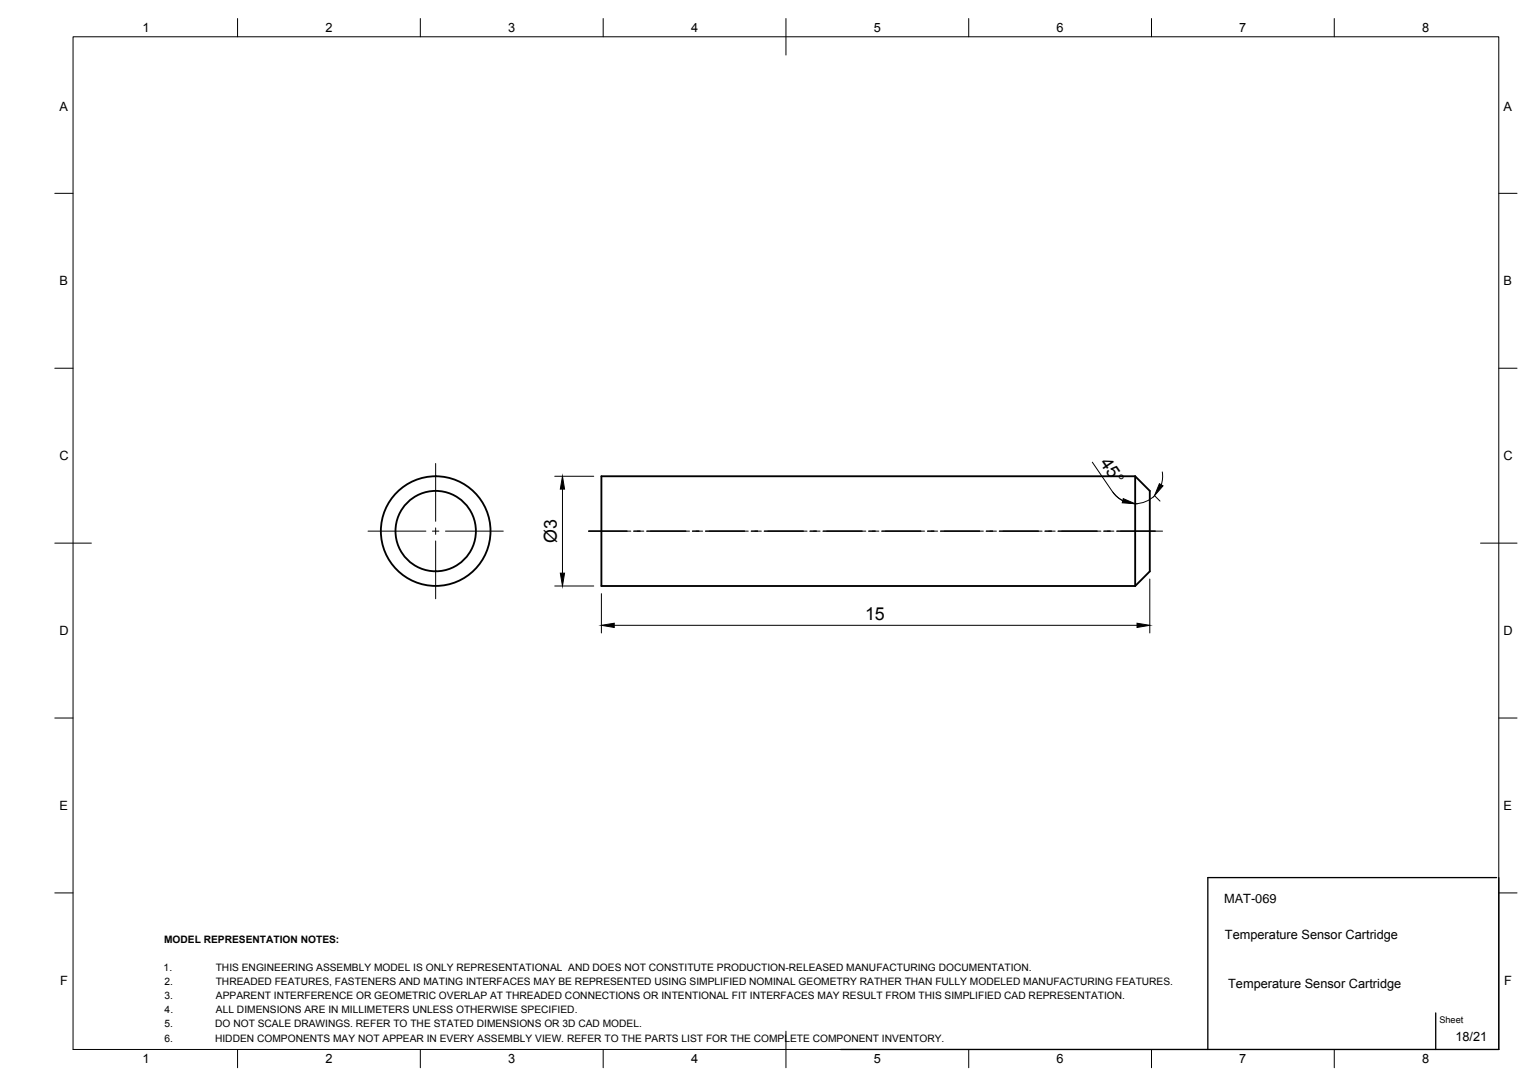
ISO-10303-21;
HEADER;
/* Generated by software containing ST-Developer
 * from STEP Tools, Inc. (www.steptools.com) 
 */

FILE_DESCRIPTION(
/* description */ ('CAx-IF Rec.Pracs.---Representation and Presentation of Product Manufa
cturing Information (PMI)---4.0---2014-10-13'),
/* implementation_level */ '2;1');

FILE_NAME(
/* name */ 'Temperature Sensor Cartridge.step',
/* time_stamp */ '2026-10-24T15:08:39-07:00',
/* author */ (''),
/* organization */ (''),
/* preprocessor_version */ 'ST-DEVELOPER v20.2',
/* originating_system */ 'Autodesk Translation Framework v15.17.0.0',
/* authorisation */ '');

FILE_SCHEMA (('AP242_MANAGED_MODEL_BASED_3D_ENGINEERING_MIM_LF { 1 0 10303 442 2 1 4 }'));
ENDSEC;

DATA;
#10=MECHANICAL_DESIGN_GEOMETRIC_PRESENTATION_REPRESENTATION('',(#835),#50081);
#654=CONICAL_SURFACE('',#10892,0.0013,0.785398163397448);
#795=SHAPE_REPRESENTATION_RELATIONSHIP('SRR','None',#50163,#815);
#815=ADVANCED_BREP_SHAPE_REPRESENTATION('',(#855),#50076);
#835=STYLED_ITEM('',(#50262),#855);
#855=MANIFOLD_SOLID_BREP('Body1',#9880);
#1083=PLANE('',#10897);
#1084=PLANE('',#10898);
#1562=FACE_OUTER_BOUND('',#2157,.T.);
#1563=FACE_OUTER_BOUND('',#2158,.T.);
#1564=FACE_OUTER_BOUND('',#2159,.T.);
#1565=FACE_OUTER_BOUND('',#2160,.T.);
#2157=EDGE_LOOP('',(#8760,#8761,#8762,#8763));
#2158=EDGE_LOOP('',(#8764,#8765,#8766,#8767));
#2159=EDGE_LOOP('',(#8768));
#2160=EDGE_LOOP('',(#8769));
#2764=LINE('',#45877,#3342);
#2765=LINE('',#45882,#3343);
#3342=VECTOR('',#13132,0.0013);
#3343=VECTOR('',#13139,0.0015);
#3730=CIRCLE('',#10893,0.00150000000001);
#3731=CIRCLE('',#10894,0.00110000000001);
#3732=CIRCLE('',#10896,0.00150000000001);
#4641=VERTEX_POINT('',#45874);
#4642=VERTEX_POINT('',#45876);
#4643=VERTEX_POINT('',#45880);
#6033=EDGE_CURVE('',#4641,#4641,#3730,.T.);
#6034=EDGE_CURVE('',#4641,#4642,#2764,.T.);
#6035=EDGE_CURVE('',#4642,#4642,#3731,.T.);
#6036=EDGE_CURVE('',#4643,#4643,#3732,.T.);
#6037=EDGE_CURVE('',#4643,#4641,#2765,.T.);
#8760=ORIENTED_EDGE('',*,*,#6033,.T.);
#8761=ORIENTED_EDGE('',*,*,#6034,.T.);
#8762=ORIENTED_EDGE('',*,*,#6035,.T.);
#8763=ORIENTED_EDGE('',*,*,#6034,.F.);
#8764=ORIENTED_EDGE('',*,*,#6036,.F.);
#8765=ORIENTED_EDGE('',*,*,#6037,.T.);
#8766=ORIENTED_EDGE('',*,*,#6033,.F.);
#8767=ORIENTED_EDGE('',*,*,#6037,.F.);
#8768=ORIENTED_EDGE('',*,*,#6035,.F.);
#8769=ORIENTED_EDGE('',*,*,#6036,.T.);
#9280=CYLINDRICAL_SURFACE('',#10895,0.0015);
#9784=ADVANCED_FACE('',(#1562),#654,.T.);
#9785=ADVANCED_FACE('',(#1563),#9280,.T.);
#9786=ADVANCED_FACE('',(#1564),#1083,.F.);
#9787=ADVANCED_FACE('',(#1565),#1084,.T.);
#9880=CLOSED_SHELL('',(#9784,#9785,#9786,#9787));
#10891=AXIS2_PLACEMENT_3D('',#45872,#13126,#13127);
#10892=AXIS2_PLACEMENT_3D('',#45873,#13128,#13129);
#10893=AXIS2_PLACEMENT_3D('',#45875,#13130,#13131);
#10894=AXIS2_PLACEMENT_3D('',#45878,#13133,#13134);
#10895=AXIS2_PLACEMENT_3D('',#45879,#13135,#13136);
#10896=AXIS2_PLACEMENT_3D('',#45881,#13137,#13138);
#10897=AXIS2_PLACEMENT_3D('',#45883,#13140,#13141);
#10898=AXIS2_PLACEMENT_3D('',#45884,#13142,#13143);
#13126=DIRECTION('axis',(0.,0.,1.));
#13127=DIRECTION('refdir',(1.,0.,0.));
#13128=DIRECTION('center_axis',(-2.42833204006769E-16,-2.41473507855972E-15,
1.));
#13129=DIRECTION('ref_axis',(0.422618261740706,0.906307787036647,2.29111895189949E-15));
#13130=DIRECTION('center_axis',(2.42833204006769E-16,2.41473507855972E-15,
-1.));
#13131=DIRECTION('ref_axis',(0.422618261740706,0.906307787036647,2.29111895189949E-15));
#13132=DIRECTION('',(0.298836238730124,0.640856382055788,-0.707106781186546));
#13133=DIRECTION('center_axis',(-2.42833204006769E-16,-2.41473507855972E-15,
1.));
#13134=DIRECTION('ref_axis',(0.422618261740706,0.906307787036647,2.29111895189949E-15));
#13135=DIRECTION('center_axis',(-2.42833204006769E-16,-2.41473507855972E-15,
1.));
#13136=DIRECTION('ref_axis',(0.422618261740706,0.906307787036647,2.29111895189949E-15));
#13137=DIRECTION('center_axis',(-2.42833204006769E-16,-2.41473507855972E-15,
1.));
#13138=DIRECTION('ref_axis',(0.422618261740706,0.906307787036647,2.29111895189949E-15));
#13139=DIRECTION('',(2.42833204006769E-16,2.41473507855972E-15,-1.));
#13140=DIRECTION('center_axis',(-2.42833204006769E-16,-2.41473507855972E-15,
1.));
#13141=DIRECTION('ref_axis',(0.422618261740706,0.906307787036647,2.29111895189949E-15));
#13142=DIRECTION('center_axis',(-2.42833204006769E-16,-2.41473507855972E-15,
1.));
#13143=DIRECTION('ref_axis',(0.422618261740706,0.906307787036647,2.29111895189949E-15));
#45872=CARTESIAN_POINT('',(0.,0.,0.));
#45873=CARTESIAN_POINT('Origin',(0.006,-0.0355287743898723,-0.0193758532865581));
#45874=CARTESIAN_POINT('',(0.00536607260738471,-0.0368882360704363,-0.0191758532865481));
#45875=CARTESIAN_POINT('Origin',(0.006,-0.0355287743898723,-0.0191758532865481));
#45876=CARTESIAN_POINT('',(0.00553511991208311,-0.0365257129556171,-0.0195758532865531));
#45877=CARTESIAN_POINT('',(0.00545059625973708,-0.0367069745130199,-0.0193758532865581));
#45878=CARTESIAN_POINT('Origin',(0.006,-0.0355287743898723,-0.0195758532865581));
#45879=CARTESIAN_POINT('Origin',(0.006,-0.0355287743898723,-0.0195758532865581));
#45880=CARTESIAN_POINT('',(0.00536607260738894,-0.0368882360704273,-0.0045758532865481));
#45881=CARTESIAN_POINT('Origin',(0.006,-0.0355287743898724,-0.0045758532865481));
#45882=CARTESIAN_POINT('',(0.00536607260738894,-0.0368882360704273,-0.0195758532865581));
#45883=CARTESIAN_POINT('Origin',(0.006,-0.0355287743898723,-0.0195758532865581));
#45884=CARTESIAN_POINT('Origin',(0.006,-0.0355287743898724,-0.0045758532865581));
#50054=UNCERTAINTY_MEASURE_WITH_UNIT(LENGTH_MEASURE(1.E-5),#50082,
'DISTANCE_ACCURACY_VALUE',
'Maximum model space distance between geometric entities at asserted c
onnectivities');
#50059=UNCERTAINTY_MEASURE_WITH_UNIT(LENGTH_MEASURE(1.E-5),#50082,
'DISTANCE_ACCURACY_VALUE',
'Maximum model space distance between geometric entities at asserted c
onnectivities');
#50076=(
GEOMETRIC_REPRESENTATION_CONTEXT(3)
GLOBAL_UNCERTAINTY_ASSIGNED_CONTEXT((#50054))
GLOBAL_UNIT_ASSIGNED_CONTEXT((#50082,#50083,#50084))
REPRESENTATION_CONTEXT('','3D')
);
#50081=(
GEOMETRIC_REPRESENTATION_CONTEXT(3)
GLOBAL_UNCERTAINTY_ASSIGNED_CONTEXT((#50059))
GLOBAL_UNIT_ASSIGNED_CONTEXT((#50082,#50083,#50084))
REPRESENTATION_CONTEXT('','3D')
);
#50082=(
LENGTH_UNIT()
NAMED_UNIT(*)
SI_UNIT($,.METRE.)
);
#50083=(
NAMED_UNIT(*)
PLANE_ANGLE_UNIT()
SI_UNIT($,.RADIAN.)
);
#50084=(
NAMED_UNIT(*)
SI_UNIT($,.STERADIAN.)
SOLID_ANGLE_UNIT()
);
#50101=SHAPE_DEFINITION_REPRESENTATION(#50122,#50163);
#50122=PRODUCT_DEFINITION_SHAPE('',$,#50185);
#50163=SHAPE_REPRESENTATION('',(#10891),#50076);
#50168=PRODUCT_DEFINITION_CONTEXT('part definition',#50233,'design');
#50185=PRODUCT_DEFINITION('Temperature Sensor Cartridge',
'Temperature Sensor Cartridge',#50206,#50168);
#50206=PRODUCT_DEFINITION_FORMATION('',$,#50251);
#50233=APPLICATION_CONTEXT('Managed model based 3d engineering');
#50234=PRODUCT_CONTEXT('part definition',#50233,'mechanical');
#50251=PRODUCT('Temperature Sensor Cartridge',
'Temperature Sensor Cartridge',
'LEGAL AND USAGE DISCLAIMER: this Data/Model is provided \X2\201C\X0\A
S IS\X2\201D\X0\ for informational and representational only. It is a 
geometric approximation and is NOT engineered, certified, or guarantee
d for dimensional accuracy, exact tolerances, or production-level prec
ision. Vendor disclaims all implied warranties including fitness for a
 particular purpose. DO NOT USE FOR DIRECT PHYSICAL MANUFACTURING, AUT
OMATED PRODUCTION, OR SAFETY-CRITICAL SYSTEMS without independent engi
neering verification and resolution of any design discrepancies.',(#50234));
#50262=PRESENTATION_STYLE_ASSIGNMENT((#50269));
#50269=SURFACE_STYLE_USAGE(.BOTH.,#50276);
#50276=SURFACE_SIDE_STYLE('',(#50283));
#50283=SURFACE_STYLE_FILL_AREA(#50290);
#50290=FILL_AREA_STYLE('Opaque(48,59,150)',(#50297));
#50297=FILL_AREA_STYLE_COLOUR('Opaque(48,59,150)',#50304);
#50304=COLOUR_RGB('Opaque(48,59,150)',0.188235294117647,0.231372549019608,
0.588235294117647);
ENDSEC;
END-ISO-10303-21;
